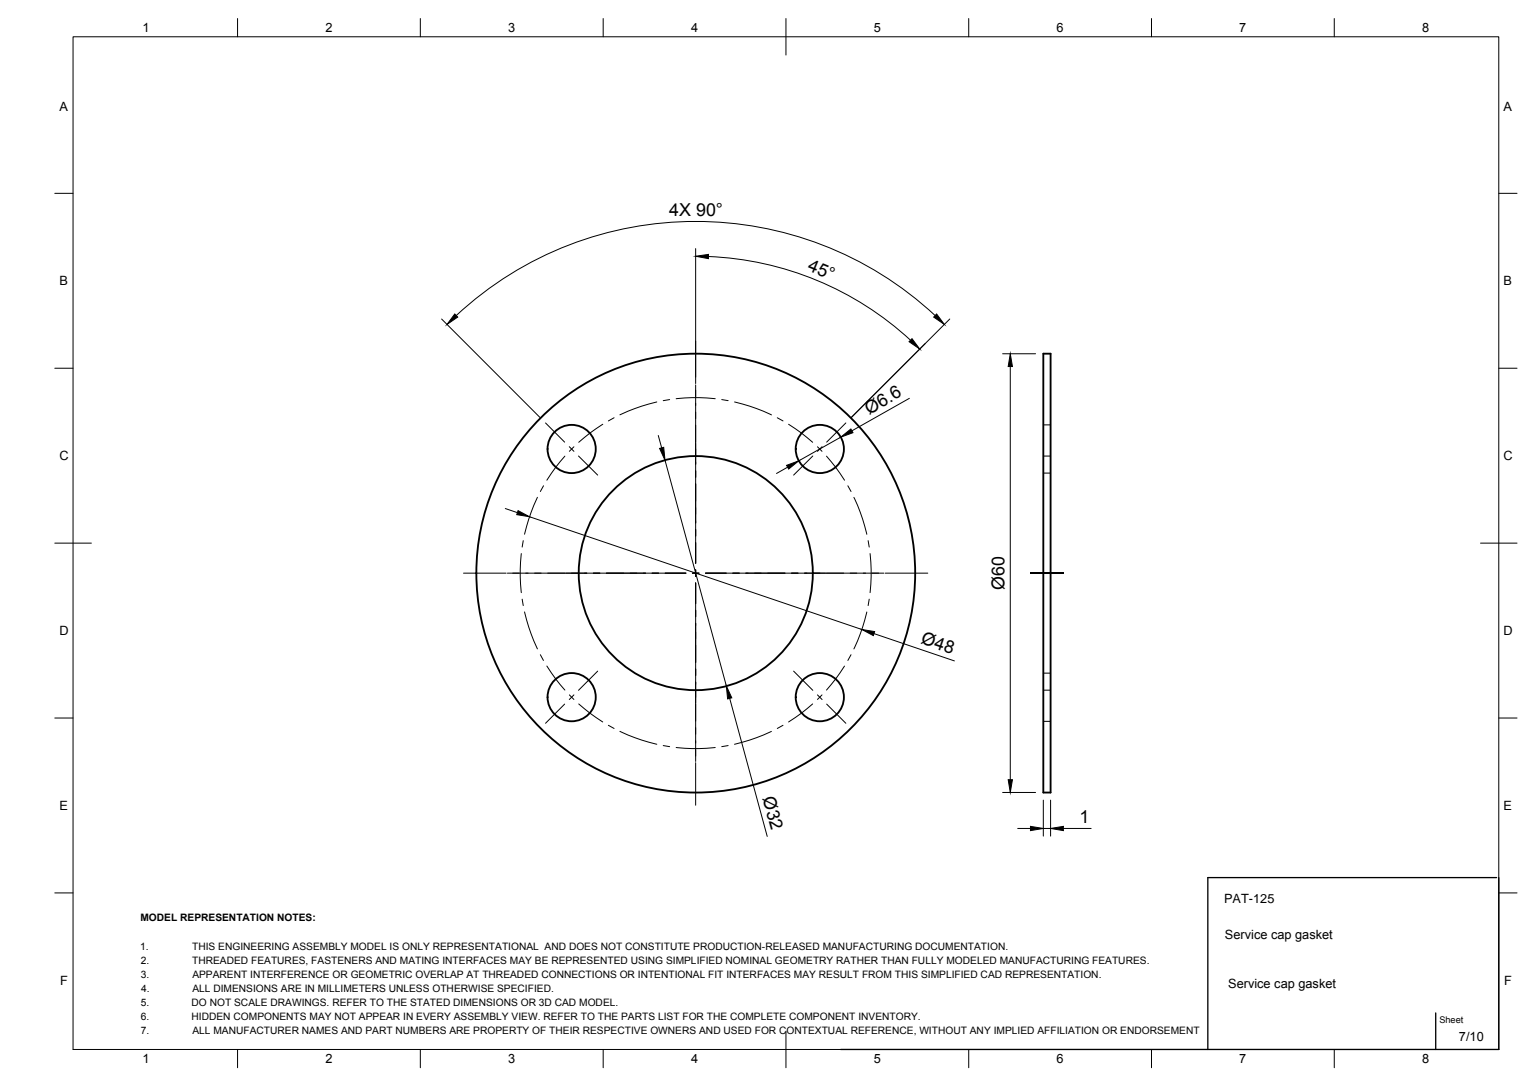
ISO-10303-21;
HEADER;
/* Generated by software containing ST-Developer
 * from STEP Tools, Inc. (www.steptools.com) 
 */

FILE_DESCRIPTION(
/* description */ ('Y-strainer with drain'),
/* implementation_level */ '2;1');

FILE_NAME(
/* name */ 'Service cap gasket.step',
/* time_stamp */ '2026-10-28T00:41:55-07:00',
/* author */ (''),
/* organization */ (''),
/* preprocessor_version */ 'ST-DEVELOPER v20.2',
/* originating_system */ 'Autodesk Translation Framework v15.17.0.0',
/* authorisation */ '');

FILE_SCHEMA (('AUTOMOTIVE_DESIGN { 1 0 10303 214 3 1 1 }'));
ENDSEC;

DATA;
#10=MECHANICAL_DESIGN_GEOMETRIC_PRESENTATION_REPRESENTATION('',(#97),#8864);
#79=SHAPE_REPRESENTATION_RELATIONSHIP('SRR','None',#8911,#88);
#88=ADVANCED_BREP_SHAPE_REPRESENTATION('',(#106),#8859);
#97=STYLED_ITEM('',(#9019),#106);
#106=MANIFOLD_SOLID_BREP('Body1',#3387);
#429=FACE_BOUND('',#881,.T.);
#430=FACE_BOUND('',#882,.T.);
#431=FACE_BOUND('',#883,.T.);
#432=FACE_BOUND('',#884,.T.);
#433=FACE_BOUND('',#885,.T.);
#434=FACE_BOUND('',#887,.T.);
#435=FACE_BOUND('',#888,.T.);
#436=FACE_BOUND('',#889,.T.);
#437=FACE_BOUND('',#890,.T.);
#438=FACE_BOUND('',#891,.T.);
#485=PLANE('',#3667);
#486=PLANE('',#3668);
#612=FACE_OUTER_BOUND('',#874,.T.);
#613=FACE_OUTER_BOUND('',#875,.T.);
#614=FACE_OUTER_BOUND('',#876,.T.);
#615=FACE_OUTER_BOUND('',#877,.T.);
#616=FACE_OUTER_BOUND('',#878,.T.);
#617=FACE_OUTER_BOUND('',#879,.T.);
#618=FACE_OUTER_BOUND('',#880,.T.);
#619=FACE_OUTER_BOUND('',#886,.T.);
#874=EDGE_LOOP('',(#2894,#2895,#2896,#2897));
#875=EDGE_LOOP('',(#2898,#2899,#2900,#2901));
#876=EDGE_LOOP('',(#2902,#2903,#2904,#2905));
#877=EDGE_LOOP('',(#2906,#2907,#2908,#2909));
#878=EDGE_LOOP('',(#2910,#2911,#2912,#2913));
#879=EDGE_LOOP('',(#2914,#2915,#2916,#2917));
#880=EDGE_LOOP('',(#2918));
#881=EDGE_LOOP('',(#2919));
#882=EDGE_LOOP('',(#2920));
#883=EDGE_LOOP('',(#2921));
#884=EDGE_LOOP('',(#2922));
#885=EDGE_LOOP('',(#2923));
#886=EDGE_LOOP('',(#2924));
#887=EDGE_LOOP('',(#2925));
#888=EDGE_LOOP('',(#2926));
#889=EDGE_LOOP('',(#2927));
#890=EDGE_LOOP('',(#2928));
#891=EDGE_LOOP('',(#2929));
#1045=LINE('',#8564,#1208);
#1046=LINE('',#8570,#1209);
#1047=LINE('',#8576,#1210);
#1048=LINE('',#8582,#1211);
#1049=LINE('',#8588,#1212);
#1050=LINE('',#8594,#1213);
#1208=VECTOR('',#4171,0.33);
#1209=VECTOR('',#4178,0.33);
#1210=VECTOR('',#4185,0.33);
#1211=VECTOR('',#4192,0.33);
#1212=VECTOR('',#4199,1.6);
#1213=VECTOR('',#4206,3.);
#1335=CIRCLE('',#3650,0.33);
#1336=CIRCLE('',#3651,0.33);
#1337=CIRCLE('',#3653,0.33);
#1338=CIRCLE('',#3654,0.33);
#1339=CIRCLE('',#3656,0.33);
#1340=CIRCLE('',#3657,0.33);
#1341=CIRCLE('',#3659,0.33);
#1342=CIRCLE('',#3660,0.33);
#1343=CIRCLE('',#3662,1.6);
#1344=CIRCLE('',#3663,1.6);
#1345=CIRCLE('',#3665,3.);
#1346=CIRCLE('',#3666,3.);
#1641=VERTEX_POINT('',#8561);
#1642=VERTEX_POINT('',#8563);
#1643=VERTEX_POINT('',#8567);
#1644=VERTEX_POINT('',#8569);
#1645=VERTEX_POINT('',#8573);
#1646=VERTEX_POINT('',#8575);
#1647=VERTEX_POINT('',#8579);
#1648=VERTEX_POINT('',#8581);
#1649=VERTEX_POINT('',#8585);
#1650=VERTEX_POINT('',#8587);
#1651=VERTEX_POINT('',#8591);
#1652=VERTEX_POINT('',#8593);
#2071=EDGE_CURVE('',#1641,#1641,#1335,.T.);
#2072=EDGE_CURVE('',#1641,#1642,#1045,.T.);
#2073=EDGE_CURVE('',#1642,#1642,#1336,.T.);
#2074=EDGE_CURVE('',#1643,#1643,#1337,.T.);
#2075=EDGE_CURVE('',#1643,#1644,#1046,.T.);
#2076=EDGE_CURVE('',#1644,#1644,#1338,.T.);
#2077=EDGE_CURVE('',#1645,#1645,#1339,.T.);
#2078=EDGE_CURVE('',#1645,#1646,#1047,.T.);
#2079=EDGE_CURVE('',#1646,#1646,#1340,.T.);
#2080=EDGE_CURVE('',#1647,#1647,#1341,.T.);
#2081=EDGE_CURVE('',#1647,#1648,#1048,.T.);
#2082=EDGE_CURVE('',#1648,#1648,#1342,.T.);
#2083=EDGE_CURVE('',#1649,#1649,#1343,.T.);
#2084=EDGE_CURVE('',#1649,#1650,#1049,.T.);
#2085=EDGE_CURVE('',#1650,#1650,#1344,.T.);
#2086=EDGE_CURVE('',#1651,#1651,#1345,.T.);
#2087=EDGE_CURVE('',#1651,#1652,#1050,.T.);
#2088=EDGE_CURVE('',#1652,#1652,#1346,.T.);
#2894=ORIENTED_EDGE('',*,*,#2071,.F.);
#2895=ORIENTED_EDGE('',*,*,#2072,.T.);
#2896=ORIENTED_EDGE('',*,*,#2073,.F.);
#2897=ORIENTED_EDGE('',*,*,#2072,.F.);
#2898=ORIENTED_EDGE('',*,*,#2074,.F.);
#2899=ORIENTED_EDGE('',*,*,#2075,.T.);
#2900=ORIENTED_EDGE('',*,*,#2076,.F.);
#2901=ORIENTED_EDGE('',*,*,#2075,.F.);
#2902=ORIENTED_EDGE('',*,*,#2077,.F.);
#2903=ORIENTED_EDGE('',*,*,#2078,.T.);
#2904=ORIENTED_EDGE('',*,*,#2079,.F.);
#2905=ORIENTED_EDGE('',*,*,#2078,.F.);
#2906=ORIENTED_EDGE('',*,*,#2080,.F.);
#2907=ORIENTED_EDGE('',*,*,#2081,.T.);
#2908=ORIENTED_EDGE('',*,*,#2082,.F.);
#2909=ORIENTED_EDGE('',*,*,#2081,.F.);
#2910=ORIENTED_EDGE('',*,*,#2083,.F.);
#2911=ORIENTED_EDGE('',*,*,#2084,.T.);
#2912=ORIENTED_EDGE('',*,*,#2085,.T.);
#2913=ORIENTED_EDGE('',*,*,#2084,.F.);
#2914=ORIENTED_EDGE('',*,*,#2086,.F.);
#2915=ORIENTED_EDGE('',*,*,#2087,.T.);
#2916=ORIENTED_EDGE('',*,*,#2088,.T.);
#2917=ORIENTED_EDGE('',*,*,#2087,.F.);
#2918=ORIENTED_EDGE('',*,*,#2086,.T.);
#2919=ORIENTED_EDGE('',*,*,#2083,.T.);
#2920=ORIENTED_EDGE('',*,*,#2082,.T.);
#2921=ORIENTED_EDGE('',*,*,#2079,.T.);
#2922=ORIENTED_EDGE('',*,*,#2076,.T.);
#2923=ORIENTED_EDGE('',*,*,#2073,.T.);
#2924=ORIENTED_EDGE('',*,*,#2088,.F.);
#2925=ORIENTED_EDGE('',*,*,#2085,.F.);
#2926=ORIENTED_EDGE('',*,*,#2080,.T.);
#2927=ORIENTED_EDGE('',*,*,#2077,.T.);
#2928=ORIENTED_EDGE('',*,*,#2074,.T.);
#2929=ORIENTED_EDGE('',*,*,#2071,.T.);
#3212=CYLINDRICAL_SURFACE('',#3649,0.33);
#3213=CYLINDRICAL_SURFACE('',#3652,0.33);
#3214=CYLINDRICAL_SURFACE('',#3655,0.33);
#3215=CYLINDRICAL_SURFACE('',#3658,0.33);
#3216=CYLINDRICAL_SURFACE('',#3661,1.6);
#3217=CYLINDRICAL_SURFACE('',#3664,3.);
#3323=ADVANCED_FACE('',(#612),#3212,.F.);
#3324=ADVANCED_FACE('',(#613),#3213,.F.);
#3325=ADVANCED_FACE('',(#614),#3214,.F.);
#3326=ADVANCED_FACE('',(#615),#3215,.F.);
#3327=ADVANCED_FACE('',(#616),#3216,.F.);
#3328=ADVANCED_FACE('',(#617),#3217,.T.);
#3329=ADVANCED_FACE('',(#618,#429,#430,#431,#432,#433),#485,.T.);
#3330=ADVANCED_FACE('',(#619,#434,#435,#436,#437,#438),#486,.F.);
#3387=CLOSED_SHELL('',(#3323,#3324,#3325,#3326,#3327,#3328,#3329,#3330));
#3648=AXIS2_PLACEMENT_3D('',#8559,#4165,#4166);
#3649=AXIS2_PLACEMENT_3D('',#8560,#4167,#4168);
#3650=AXIS2_PLACEMENT_3D('',#8562,#4169,#4170);
#3651=AXIS2_PLACEMENT_3D('',#8565,#4172,#4173);
#3652=AXIS2_PLACEMENT_3D('',#8566,#4174,#4175);
#3653=AXIS2_PLACEMENT_3D('',#8568,#4176,#4177);
#3654=AXIS2_PLACEMENT_3D('',#8571,#4179,#4180);
#3655=AXIS2_PLACEMENT_3D('',#8572,#4181,#4182);
#3656=AXIS2_PLACEMENT_3D('',#8574,#4183,#4184);
#3657=AXIS2_PLACEMENT_3D('',#8577,#4186,#4187);
#3658=AXIS2_PLACEMENT_3D('',#8578,#4188,#4189);
#3659=AXIS2_PLACEMENT_3D('',#8580,#4190,#4191);
#3660=AXIS2_PLACEMENT_3D('',#8583,#4193,#4194);
#3661=AXIS2_PLACEMENT_3D('',#8584,#4195,#4196);
#3662=AXIS2_PLACEMENT_3D('',#8586,#4197,#4198);
#3663=AXIS2_PLACEMENT_3D('',#8589,#4200,#4201);
#3664=AXIS2_PLACEMENT_3D('',#8590,#4202,#4203);
#3665=AXIS2_PLACEMENT_3D('',#8592,#4204,#4205);
#3666=AXIS2_PLACEMENT_3D('',#8595,#4207,#4208);
#3667=AXIS2_PLACEMENT_3D('',#8596,#4209,#4210);
#3668=AXIS2_PLACEMENT_3D('',#8597,#4211,#4212);
#4165=DIRECTION('axis',(0.,0.,1.));
#4166=DIRECTION('refdir',(1.,0.,0.));
#4167=DIRECTION('center_axis',(0.707106781186548,0.,-0.707106781186547));
#4168=DIRECTION('ref_axis',(-0.707106781186547,0.,-0.707106781186548));
#4169=DIRECTION('center_axis',(0.707106781186548,0.,-0.707106781186547));
#4170=DIRECTION('ref_axis',(-0.707106781186547,0.,-0.707106781186548));
#4171=DIRECTION('',(0.707106781186548,0.,-0.707106781186547));
#4172=DIRECTION('center_axis',(-0.707106781186548,0.,0.707106781186547));
#4173=DIRECTION('ref_axis',(-0.707106781186547,0.,-0.707106781186548));
#4174=DIRECTION('center_axis',(0.707106781186548,0.,-0.707106781186547));
#4175=DIRECTION('ref_axis',(-0.707106781186547,0.,-0.707106781186548));
#4176=DIRECTION('center_axis',(0.707106781186548,0.,-0.707106781186547));
#4177=DIRECTION('ref_axis',(-0.707106781186547,0.,-0.707106781186548));
#4178=DIRECTION('',(0.707106781186548,0.,-0.707106781186547));
#4179=DIRECTION('center_axis',(-0.707106781186548,0.,0.707106781186547));
#4180=DIRECTION('ref_axis',(-0.707106781186547,0.,-0.707106781186548));
#4181=DIRECTION('center_axis',(0.707106781186548,0.,-0.707106781186547));
#4182=DIRECTION('ref_axis',(-0.707106781186547,0.,-0.707106781186548));
#4183=DIRECTION('center_axis',(0.707106781186548,0.,-0.707106781186547));
#4184=DIRECTION('ref_axis',(-0.707106781186547,0.,-0.707106781186548));
#4185=DIRECTION('',(0.707106781186548,0.,-0.707106781186547));
#4186=DIRECTION('center_axis',(-0.707106781186548,0.,0.707106781186547));
#4187=DIRECTION('ref_axis',(-0.707106781186547,0.,-0.707106781186548));
#4188=DIRECTION('center_axis',(0.707106781186548,0.,-0.707106781186547));
#4189=DIRECTION('ref_axis',(-0.707106781186547,0.,-0.707106781186548));
#4190=DIRECTION('center_axis',(0.707106781186548,0.,-0.707106781186547));
#4191=DIRECTION('ref_axis',(-0.707106781186547,0.,-0.707106781186548));
#4192=DIRECTION('',(0.707106781186548,0.,-0.707106781186547));
#4193=DIRECTION('center_axis',(-0.707106781186548,0.,0.707106781186547));
#4194=DIRECTION('ref_axis',(-0.707106781186547,0.,-0.707106781186548));
#4195=DIRECTION('center_axis',(0.707106781186548,0.,-0.707106781186547));
#4196=DIRECTION('ref_axis',(-0.707106781186547,0.,-0.707106781186548));
#4197=DIRECTION('center_axis',(-0.707106781186548,0.,0.707106781186547));
#4198=DIRECTION('ref_axis',(-0.707106781186547,0.,-0.707106781186548));
#4199=DIRECTION('',(-0.707106781186548,0.,0.707106781186547));
#4200=DIRECTION('center_axis',(-0.707106781186548,0.,0.707106781186547));
#4201=DIRECTION('ref_axis',(-0.707106781186547,0.,-0.707106781186548));
#4202=DIRECTION('center_axis',(0.707106781186548,0.,-0.707106781186547));
#4203=DIRECTION('ref_axis',(-0.707106781186547,0.,-0.707106781186548));
#4204=DIRECTION('center_axis',(0.707106781186548,0.,-0.707106781186547));
#4205=DIRECTION('ref_axis',(-0.707106781186547,0.,-0.707106781186548));
#4206=DIRECTION('',(-0.707106781186548,0.,0.707106781186547));
#4207=DIRECTION('center_axis',(0.707106781186548,0.,-0.707106781186547));
#4208=DIRECTION('ref_axis',(-0.707106781186547,0.,-0.707106781186548));
#4209=DIRECTION('center_axis',(0.707106781186548,0.,-0.707106781186547));
#4210=DIRECTION('ref_axis',(-0.707106781186547,0.,-0.707106781186548));
#4211=DIRECTION('center_axis',(0.707106781186548,0.,-0.707106781186547));
#4212=DIRECTION('ref_axis',(-0.707106781186547,0.,-0.707106781186548));
#8559=CARTESIAN_POINT('',(0.,0.,0.));
#8560=CARTESIAN_POINT('Origin',(5.07903679018718,-1.69705627484771,3.32096320981282));
#8561=CARTESIAN_POINT('',(5.38309270609739,-1.69705627484771,3.48359776948573));
#8562=CARTESIAN_POINT('Origin',(5.14974746830583,-1.69705627484771,3.25025253169417));
#8563=CARTESIAN_POINT('',(5.45380338421605,-1.69705627484771,3.41288709136707));
#8564=CARTESIAN_POINT('',(5.31238202797874,-1.69705627484771,3.55430844760438));
#8565=CARTESIAN_POINT('Origin',(5.22045814642449,-1.69705627484771,3.17954185357551));
#8566=CARTESIAN_POINT('Origin',(5.07903679018718,1.69705627484771,3.32096320981282));
#8567=CARTESIAN_POINT('',(5.38309270609739,1.69705627484771,3.48359776948573));
#8568=CARTESIAN_POINT('Origin',(5.14974746830583,1.69705627484771,3.25025253169417));
#8569=CARTESIAN_POINT('',(5.45380338421605,1.69705627484771,3.41288709136707));
#8570=CARTESIAN_POINT('',(5.31238202797874,1.69705627484771,3.55430844760438));
#8571=CARTESIAN_POINT('Origin',(5.22045814642449,1.69705627484771,3.17954185357551));
#8572=CARTESIAN_POINT('Origin',(2.67903679018718,1.69705627484771,0.920963209812822));
#8573=CARTESIAN_POINT('',(2.98309270609739,1.69705627484771,1.08359776948573));
#8574=CARTESIAN_POINT('Origin',(2.74974746830583,1.69705627484771,0.850252531694168));
#8575=CARTESIAN_POINT('',(3.05380338421605,1.69705627484771,1.01288709136707));
#8576=CARTESIAN_POINT('',(2.91238202797874,1.69705627484771,1.15430844760438));
#8577=CARTESIAN_POINT('Origin',(2.82045814642449,1.69705627484771,0.779541853575513));
#8578=CARTESIAN_POINT('Origin',(2.67903679018718,-1.69705627484771,0.920963209812822));
#8579=CARTESIAN_POINT('',(2.98309270609739,-1.69705627484771,1.08359776948573));
#8580=CARTESIAN_POINT('Origin',(2.74974746830583,-1.69705627484771,0.850252531694168));
#8581=CARTESIAN_POINT('',(3.05380338421605,-1.69705627484771,1.01288709136707));
#8582=CARTESIAN_POINT('',(2.91238202797874,-1.69705627484771,1.15430844760438));
#8583=CARTESIAN_POINT('Origin',(2.82045814642449,-1.69705627484771,0.779541853575513));
#8584=CARTESIAN_POINT('Origin',(3.94974746830583,0.,2.05025253169417));
#8585=CARTESIAN_POINT('',(5.15182899632296,-1.95943487863577E-16,3.11091270347399));
#8586=CARTESIAN_POINT('Origin',(4.02045814642449,0.,1.97954185357551));
#8587=CARTESIAN_POINT('',(5.08111831820431,-1.95943487863577E-16,3.18162338159264));
#8588=CARTESIAN_POINT('',(5.08111831820431,-1.95943487863577E-16,3.18162338159264));
#8589=CARTESIAN_POINT('Origin',(3.94974746830583,0.,2.05025253169417));
#8590=CARTESIAN_POINT('Origin',(3.94974746830583,0.,2.05025253169417));
#8591=CARTESIAN_POINT('',(6.14177848998413,-3.67394039744206E-16,4.10086219713516));
#8592=CARTESIAN_POINT('Origin',(4.02045814642449,0.,1.97954185357551));
#8593=CARTESIAN_POINT('',(6.07106781186548,-3.67394039744206E-16,4.17157287525381));
#8594=CARTESIAN_POINT('',(6.07106781186548,-3.67394039744206E-16,4.17157287525381));
#8595=CARTESIAN_POINT('Origin',(3.94974746830583,0.,2.05025253169417));
#8596=CARTESIAN_POINT('Origin',(4.02045814642449,0.,1.97954185357551));
#8597=CARTESIAN_POINT('Origin',(3.94974746830583,0.,2.05025253169417));
#8847=UNCERTAINTY_MEASURE_WITH_UNIT(LENGTH_MEASURE(0.001),#8865,
'DISTANCE_ACCURACY_VALUE',
'Maximum model space distance between geometric entities at asserted c
onnectivities');
#8852=UNCERTAINTY_MEASURE_WITH_UNIT(LENGTH_MEASURE(0.001),#8865,
'DISTANCE_ACCURACY_VALUE',
'Maximum model space distance between geometric entities at asserted c
onnectivities');
#8859=(
GEOMETRIC_REPRESENTATION_CONTEXT(3)
GLOBAL_UNCERTAINTY_ASSIGNED_CONTEXT((#8847))
GLOBAL_UNIT_ASSIGNED_CONTEXT((#8865,#8867,#8868))
REPRESENTATION_CONTEXT('','3D')
);
#8864=(
GEOMETRIC_REPRESENTATION_CONTEXT(3)
GLOBAL_UNCERTAINTY_ASSIGNED_CONTEXT((#8852))
GLOBAL_UNIT_ASSIGNED_CONTEXT((#8865,#8867,#8868))
REPRESENTATION_CONTEXT('','3D')
);
#8865=(
LENGTH_UNIT()
NAMED_UNIT(*)
SI_UNIT(.CENTI.,.METRE.)
);
#8867=(
NAMED_UNIT(*)
PLANE_ANGLE_UNIT()
SI_UNIT($,.RADIAN.)
);
#8868=(
NAMED_UNIT(*)
SI_UNIT($,.STERADIAN.)
SOLID_ANGLE_UNIT()
);
#8875=SHAPE_DEFINITION_REPRESENTATION(#8886,#8911);
#8886=PRODUCT_DEFINITION_SHAPE('',$,#8923);
#8911=SHAPE_REPRESENTATION('',(#3648),#8859);
#8916=PRODUCT_DEFINITION_CONTEXT('part definition',#8951,'design');
#8923=PRODUCT_DEFINITION('Service cap gasket','Service cap gasket',#8934,
#8916);
#8934=PRODUCT_DEFINITION_FORMATION('',$,#8959);
#8951=APPLICATION_CONTEXT(
'Core Data for Automotive Mechanical Design Process');
#8952=PRODUCT_CONTEXT('part definition',#8951,'mechanical');
#8959=PRODUCT('Service cap gasket','Service cap gasket',
'Service cap gasket',(#8952));
#9013=COLOUR_RGB('Light Blue',0.38,0.62,0.78);
#9014=FILL_AREA_STYLE_COLOUR('',#9013);
#9015=FILL_AREA_STYLE('',(#9014));
#9016=SURFACE_STYLE_FILL_AREA(#9015);
#9017=SURFACE_SIDE_STYLE('',(#9016));
#9018=SURFACE_STYLE_USAGE(.BOTH.,#9017);
#9019=PRESENTATION_STYLE_ASSIGNMENT((#9018));
ENDSEC;
END-ISO-10303-21;
